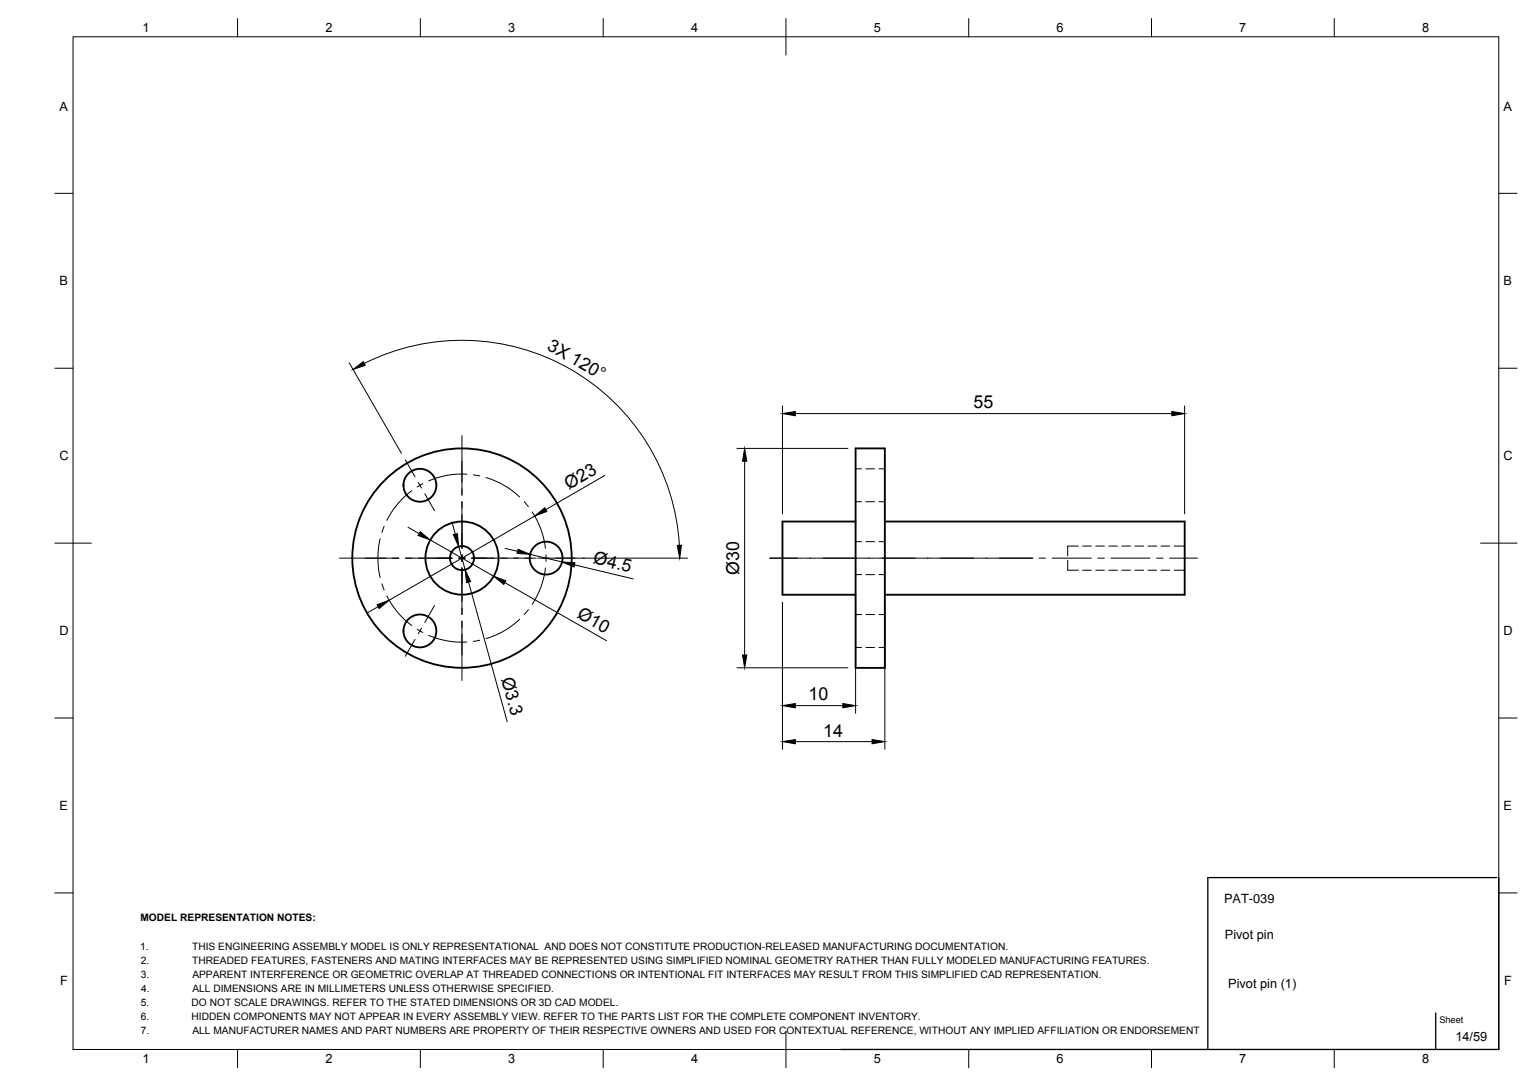
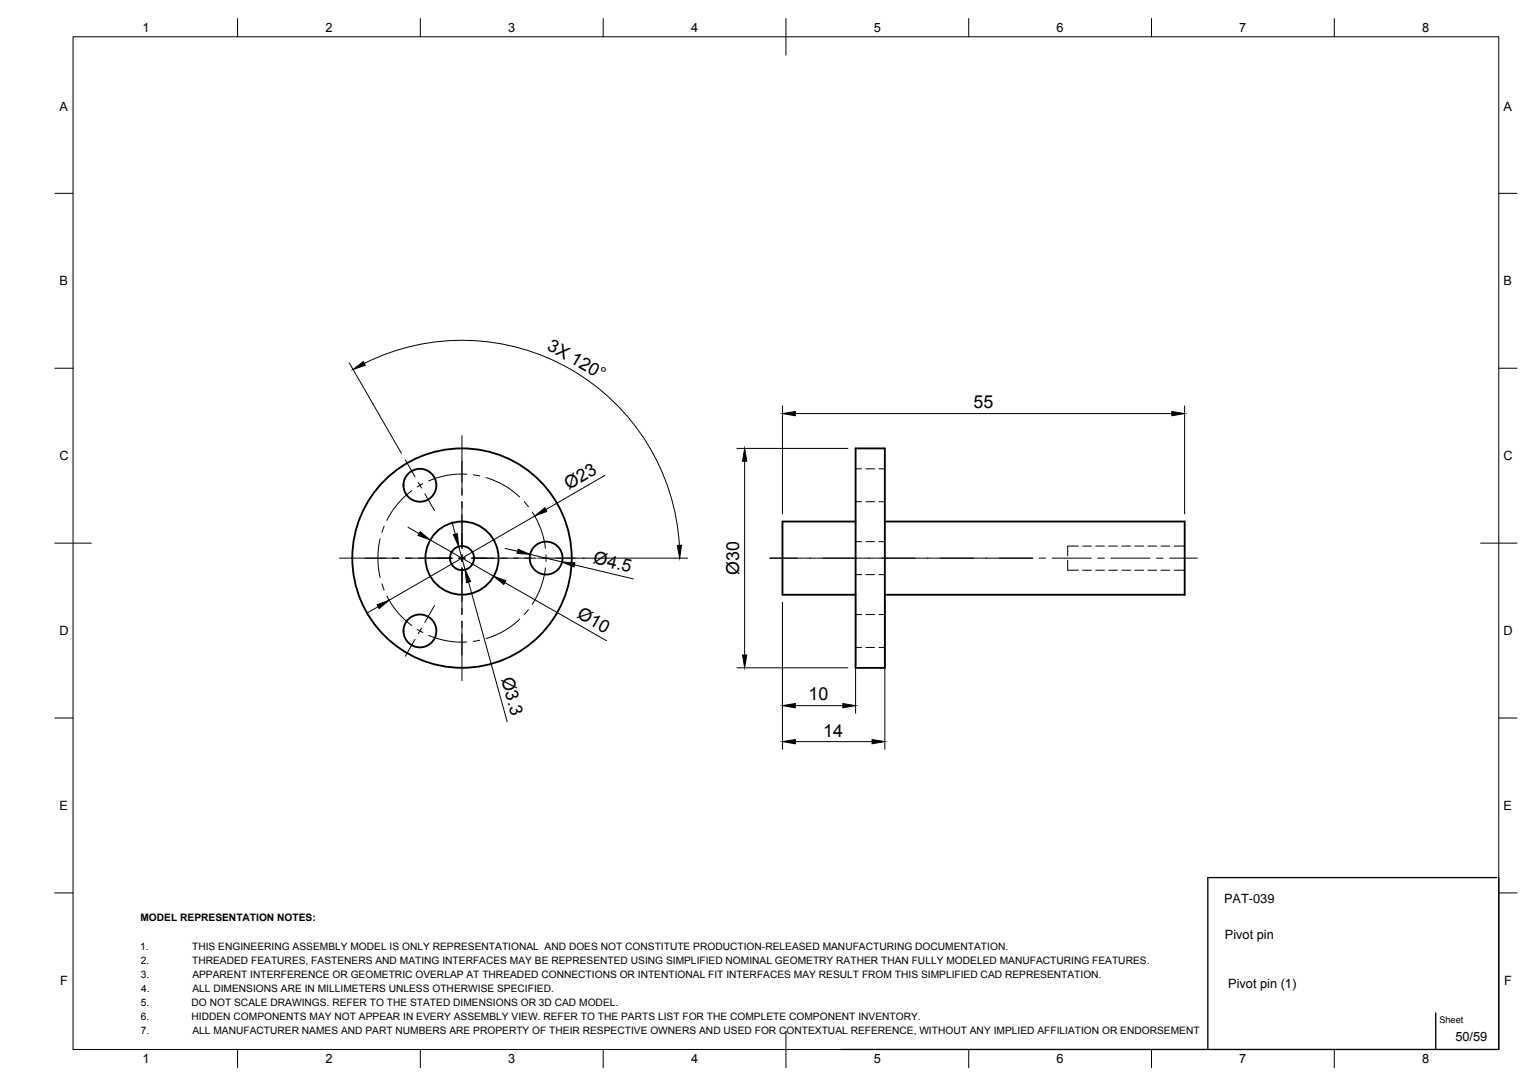
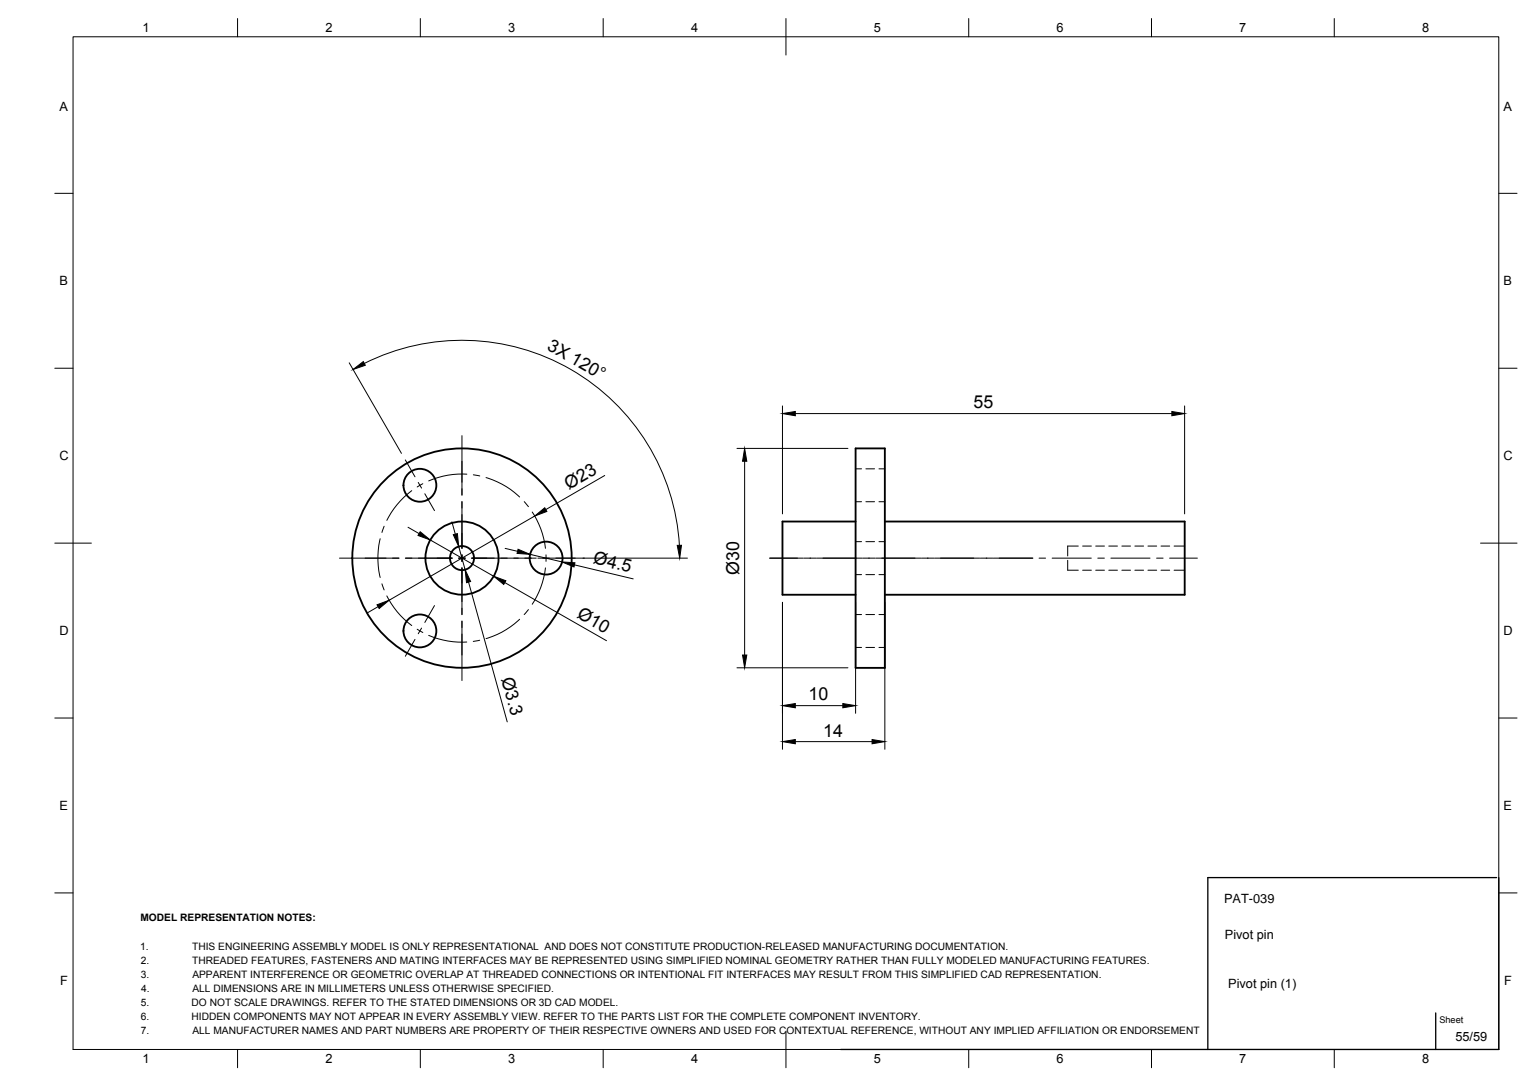
ISO-10303-21;
HEADER;
/* Generated by software containing ST-Developer
 * from STEP Tools, Inc. (www.steptools.com) 
 */

FILE_DESCRIPTION(
/* description */ ('Four-bar parallelogram arm'),
/* implementation_level */ '2;1');

FILE_NAME(
/* name */ 'Pivot pin (1).step',
/* time_stamp */ '2026-10-28T03:24:55-07:00',
/* author */ (''),
/* organization */ (''),
/* preprocessor_version */ 'ST-DEVELOPER v20.2',
/* originating_system */ 'Autodesk Translation Framework v15.17.0.0',
/* authorisation */ '');

FILE_SCHEMA (('AUTOMOTIVE_DESIGN { 1 0 10303 214 3 1 1 }'));
ENDSEC;

DATA;
#10=MECHANICAL_DESIGN_GEOMETRIC_PRESENTATION_REPRESENTATION('',(#669),#14512);
#561=SHAPE_REPRESENTATION_RELATIONSHIP('SRR','None',#14786,#611);
#611=ADVANCED_BREP_SHAPE_REPRESENTATION('',(#725),#14501);
#669=STYLED_ITEM('',(#15087),#725);
#725=MANIFOLD_SOLID_BREP('Body1',#7375);
#971=FACE_BOUND('',#2210,.T.);
#972=FACE_BOUND('',#2211,.T.);
#973=FACE_BOUND('',#2212,.T.);
#974=FACE_BOUND('',#2213,.T.);
#975=FACE_BOUND('',#2215,.T.);
#976=FACE_BOUND('',#2216,.T.);
#977=FACE_BOUND('',#2217,.T.);
#978=FACE_BOUND('',#2218,.T.);
#979=FACE_BOUND('',#2224,.T.);
#1164=PLANE('',#8770);
#1165=PLANE('',#8780);
#1166=PLANE('',#8783);
#1167=PLANE('',#8791);
#1168=PLANE('',#8792);
#1548=FACE_OUTER_BOUND('',#2204,.T.);
#1549=FACE_OUTER_BOUND('',#2205,.T.);
#1550=FACE_OUTER_BOUND('',#2206,.T.);
#1551=FACE_OUTER_BOUND('',#2207,.T.);
#1552=FACE_OUTER_BOUND('',#2208,.T.);
#1553=FACE_OUTER_BOUND('',#2209,.T.);
#1554=FACE_OUTER_BOUND('',#2214,.T.);
#1555=FACE_OUTER_BOUND('',#2219,.T.);
#1556=FACE_OUTER_BOUND('',#2220,.T.);
#1557=FACE_OUTER_BOUND('',#2221,.T.);
#1558=FACE_OUTER_BOUND('',#2222,.T.);
#1559=FACE_OUTER_BOUND('',#2223,.T.);
#2204=EDGE_LOOP('',(#6470,#6471,#6472,#6473));
#2205=EDGE_LOOP('',(#6474));
#2206=EDGE_LOOP('',(#6475,#6476,#6477,#6478));
#2207=EDGE_LOOP('',(#6479,#6480,#6481,#6482));
#2208=EDGE_LOOP('',(#6483,#6484,#6485,#6486));
#2209=EDGE_LOOP('',(#6487));
#2210=EDGE_LOOP('',(#6488));
#2211=EDGE_LOOP('',(#6489));
#2212=EDGE_LOOP('',(#6490));
#2213=EDGE_LOOP('',(#6491));
#2214=EDGE_LOOP('',(#6492));
#2215=EDGE_LOOP('',(#6493));
#2216=EDGE_LOOP('',(#6494));
#2217=EDGE_LOOP('',(#6495));
#2218=EDGE_LOOP('',(#6496));
#2219=EDGE_LOOP('',(#6497,#6498,#6499,#6500));
#2220=EDGE_LOOP('',(#6501,#6502,#6503,#6504));
#2221=EDGE_LOOP('',(#6505,#6506,#6507,#6508));
#2222=EDGE_LOOP('',(#6509));
#2223=EDGE_LOOP('',(#6510));
#2224=EDGE_LOOP('',(#6511));
#2652=LINE('',#14066,#3046);
#2653=LINE('',#14073,#3047);
#2654=LINE('',#14079,#3048);
#2655=LINE('',#14085,#3049);
#2656=LINE('',#14098,#3050);
#2657=LINE('',#14101,#3051);
#2658=LINE('',#14106,#3052);
#3046=VECTOR('',#10972,0.164999999999999);
#3047=VECTOR('',#10981,0.225000000000001);
#3048=VECTOR('',#10988,0.225000000000001);
#3049=VECTOR('',#10995,0.225000000000001);
#3050=VECTOR('',#11012,1.5);
#3051=VECTOR('',#11015,0.5);
#3052=VECTOR('',#11022,0.5);
#3477=CIRCLE('',#8768,0.164999999999999);
#3478=CIRCLE('',#8769,0.164999999999999);
#3479=CIRCLE('',#8772,0.225000000000001);
#3480=CIRCLE('',#8773,0.225000000000001);
#3481=CIRCLE('',#8775,0.225000000000001);
#3482=CIRCLE('',#8776,0.225000000000001);
#3483=CIRCLE('',#8778,0.225000000000001);
#3484=CIRCLE('',#8779,0.225000000000001);
#3485=CIRCLE('',#8781,1.5);
#3486=CIRCLE('',#8782,0.5);
#3487=CIRCLE('',#8784,1.5);
#3488=CIRCLE('',#8785,0.5);
#3489=CIRCLE('',#8788,0.5);
#3490=CIRCLE('',#8790,0.5);
#4045=VERTEX_POINT('',#14063);
#4046=VERTEX_POINT('',#14065);
#4047=VERTEX_POINT('',#14070);
#4048=VERTEX_POINT('',#14072);
#4049=VERTEX_POINT('',#14076);
#4050=VERTEX_POINT('',#14078);
#4051=VERTEX_POINT('',#14082);
#4052=VERTEX_POINT('',#14084);
#4053=VERTEX_POINT('',#14088);
#4054=VERTEX_POINT('',#14090);
#4055=VERTEX_POINT('',#14093);
#4056=VERTEX_POINT('',#14095);
#4057=VERTEX_POINT('',#14100);
#4058=VERTEX_POINT('',#14104);
#4866=EDGE_CURVE('',#4045,#4045,#3477,.T.);
#4867=EDGE_CURVE('',#4045,#4046,#2652,.T.);
#4868=EDGE_CURVE('',#4046,#4046,#3478,.T.);
#4869=EDGE_CURVE('',#4047,#4047,#3479,.T.);
#4870=EDGE_CURVE('',#4047,#4048,#2653,.T.);
#4871=EDGE_CURVE('',#4048,#4048,#3480,.T.);
#4872=EDGE_CURVE('',#4049,#4049,#3481,.T.);
#4873=EDGE_CURVE('',#4049,#4050,#2654,.T.);
#4874=EDGE_CURVE('',#4050,#4050,#3482,.T.);
#4875=EDGE_CURVE('',#4051,#4051,#3483,.T.);
#4876=EDGE_CURVE('',#4051,#4052,#2655,.T.);
#4877=EDGE_CURVE('',#4052,#4052,#3484,.T.);
#4878=EDGE_CURVE('',#4053,#4053,#3485,.T.);
#4879=EDGE_CURVE('',#4054,#4054,#3486,.T.);
#4880=EDGE_CURVE('',#4055,#4055,#3487,.T.);
#4881=EDGE_CURVE('',#4056,#4056,#3488,.T.);
#4882=EDGE_CURVE('',#4053,#4055,#2656,.T.);
#4883=EDGE_CURVE('',#4056,#4057,#2657,.T.);
#4884=EDGE_CURVE('',#4057,#4057,#3489,.T.);
#4885=EDGE_CURVE('',#4058,#4058,#3490,.T.);
#4886=EDGE_CURVE('',#4058,#4054,#2658,.T.);
#6470=ORIENTED_EDGE('',*,*,#4866,.F.);
#6471=ORIENTED_EDGE('',*,*,#4867,.T.);
#6472=ORIENTED_EDGE('',*,*,#4868,.T.);
#6473=ORIENTED_EDGE('',*,*,#4867,.F.);
#6474=ORIENTED_EDGE('',*,*,#4868,.F.);
#6475=ORIENTED_EDGE('',*,*,#4869,.F.);
#6476=ORIENTED_EDGE('',*,*,#4870,.T.);
#6477=ORIENTED_EDGE('',*,*,#4871,.F.);
#6478=ORIENTED_EDGE('',*,*,#4870,.F.);
#6479=ORIENTED_EDGE('',*,*,#4872,.F.);
#6480=ORIENTED_EDGE('',*,*,#4873,.T.);
#6481=ORIENTED_EDGE('',*,*,#4874,.F.);
#6482=ORIENTED_EDGE('',*,*,#4873,.F.);
#6483=ORIENTED_EDGE('',*,*,#4875,.F.);
#6484=ORIENTED_EDGE('',*,*,#4876,.T.);
#6485=ORIENTED_EDGE('',*,*,#4877,.F.);
#6486=ORIENTED_EDGE('',*,*,#4876,.F.);
#6487=ORIENTED_EDGE('',*,*,#4878,.T.);
#6488=ORIENTED_EDGE('',*,*,#4871,.T.);
#6489=ORIENTED_EDGE('',*,*,#4874,.T.);
#6490=ORIENTED_EDGE('',*,*,#4877,.T.);
#6491=ORIENTED_EDGE('',*,*,#4879,.F.);
#6492=ORIENTED_EDGE('',*,*,#4880,.F.);
#6493=ORIENTED_EDGE('',*,*,#4869,.T.);
#6494=ORIENTED_EDGE('',*,*,#4872,.T.);
#6495=ORIENTED_EDGE('',*,*,#4875,.T.);
#6496=ORIENTED_EDGE('',*,*,#4881,.F.);
#6497=ORIENTED_EDGE('',*,*,#4878,.F.);
#6498=ORIENTED_EDGE('',*,*,#4882,.T.);
#6499=ORIENTED_EDGE('',*,*,#4880,.T.);
#6500=ORIENTED_EDGE('',*,*,#4882,.F.);
#6501=ORIENTED_EDGE('',*,*,#4881,.T.);
#6502=ORIENTED_EDGE('',*,*,#4883,.T.);
#6503=ORIENTED_EDGE('',*,*,#4884,.T.);
#6504=ORIENTED_EDGE('',*,*,#4883,.F.);
#6505=ORIENTED_EDGE('',*,*,#4885,.F.);
#6506=ORIENTED_EDGE('',*,*,#4886,.T.);
#6507=ORIENTED_EDGE('',*,*,#4879,.T.);
#6508=ORIENTED_EDGE('',*,*,#4886,.F.);
#6509=ORIENTED_EDGE('',*,*,#4885,.T.);
#6510=ORIENTED_EDGE('',*,*,#4884,.F.);
#6511=ORIENTED_EDGE('',*,*,#4866,.T.);
#6874=CYLINDRICAL_SURFACE('',#8767,0.164999999999999);
#6875=CYLINDRICAL_SURFACE('',#8771,0.225000000000001);
#6876=CYLINDRICAL_SURFACE('',#8774,0.225000000000001);
#6877=CYLINDRICAL_SURFACE('',#8777,0.225000000000001);
#6878=CYLINDRICAL_SURFACE('',#8786,1.5);
#6879=CYLINDRICAL_SURFACE('',#8787,0.5);
#6880=CYLINDRICAL_SURFACE('',#8789,0.5);
#7253=ADVANCED_FACE('',(#1548),#6874,.F.);
#7254=ADVANCED_FACE('',(#1549),#1164,.F.);
#7255=ADVANCED_FACE('',(#1550),#6875,.F.);
#7256=ADVANCED_FACE('',(#1551),#6876,.F.);
#7257=ADVANCED_FACE('',(#1552),#6877,.F.);
#7258=ADVANCED_FACE('',(#1553,#971,#972,#973,#974),#1165,.T.);
#7259=ADVANCED_FACE('',(#1554,#975,#976,#977,#978),#1166,.F.);
#7260=ADVANCED_FACE('',(#1555),#6878,.T.);
#7261=ADVANCED_FACE('',(#1556),#6879,.T.);
#7262=ADVANCED_FACE('',(#1557),#6880,.T.);
#7263=ADVANCED_FACE('',(#1558),#1167,.T.);
#7264=ADVANCED_FACE('',(#1559,#979),#1168,.F.);
#7375=CLOSED_SHELL('',(#7253,#7254,#7255,#7256,#7257,#7258,#7259,#7260,
#7261,#7262,#7263,#7264));
#8766=AXIS2_PLACEMENT_3D('',#14061,#10966,#10967);
#8767=AXIS2_PLACEMENT_3D('',#14062,#10968,#10969);
#8768=AXIS2_PLACEMENT_3D('',#14064,#10970,#10971);
#8769=AXIS2_PLACEMENT_3D('',#14067,#10973,#10974);
#8770=AXIS2_PLACEMENT_3D('',#14068,#10975,#10976);
#8771=AXIS2_PLACEMENT_3D('',#14069,#10977,#10978);
#8772=AXIS2_PLACEMENT_3D('',#14071,#10979,#10980);
#8773=AXIS2_PLACEMENT_3D('',#14074,#10982,#10983);
#8774=AXIS2_PLACEMENT_3D('',#14075,#10984,#10985);
#8775=AXIS2_PLACEMENT_3D('',#14077,#10986,#10987);
#8776=AXIS2_PLACEMENT_3D('',#14080,#10989,#10990);
#8777=AXIS2_PLACEMENT_3D('',#14081,#10991,#10992);
#8778=AXIS2_PLACEMENT_3D('',#14083,#10993,#10994);
#8779=AXIS2_PLACEMENT_3D('',#14086,#10996,#10997);
#8780=AXIS2_PLACEMENT_3D('',#14087,#10998,#10999);
#8781=AXIS2_PLACEMENT_3D('',#14089,#11000,#11001);
#8782=AXIS2_PLACEMENT_3D('',#14091,#11002,#11003);
#8783=AXIS2_PLACEMENT_3D('',#14092,#11004,#11005);
#8784=AXIS2_PLACEMENT_3D('',#14094,#11006,#11007);
#8785=AXIS2_PLACEMENT_3D('',#14096,#11008,#11009);
#8786=AXIS2_PLACEMENT_3D('',#14097,#11010,#11011);
#8787=AXIS2_PLACEMENT_3D('',#14099,#11013,#11014);
#8788=AXIS2_PLACEMENT_3D('',#14102,#11016,#11017);
#8789=AXIS2_PLACEMENT_3D('',#14103,#11018,#11019);
#8790=AXIS2_PLACEMENT_3D('',#14105,#11020,#11021);
#8791=AXIS2_PLACEMENT_3D('',#14107,#11023,#11024);
#8792=AXIS2_PLACEMENT_3D('',#14108,#11025,#11026);
#10966=DIRECTION('axis',(0.,0.,1.));
#10967=DIRECTION('refdir',(1.,0.,0.));
#10968=DIRECTION('center_axis',(0.,1.,0.));
#10969=DIRECTION('ref_axis',(1.,0.,0.));
#10970=DIRECTION('center_axis',(0.,1.,0.));
#10971=DIRECTION('ref_axis',(1.,0.,0.));
#10972=DIRECTION('',(0.,1.,0.));
#10973=DIRECTION('center_axis',(0.,1.,0.));
#10974=DIRECTION('ref_axis',(1.,0.,0.));
#10975=DIRECTION('center_axis',(0.,1.,0.));
#10976=DIRECTION('ref_axis',(1.,0.,0.));
#10977=DIRECTION('center_axis',(0.,1.,0.));
#10978=DIRECTION('ref_axis',(1.,0.,0.));
#10979=DIRECTION('center_axis',(0.,1.,0.));
#10980=DIRECTION('ref_axis',(1.,0.,0.));
#10981=DIRECTION('',(0.,1.,0.));
#10982=DIRECTION('center_axis',(0.,-1.,0.));
#10983=DIRECTION('ref_axis',(1.,0.,0.));
#10984=DIRECTION('center_axis',(0.,1.,0.));
#10985=DIRECTION('ref_axis',(1.,0.,0.));
#10986=DIRECTION('center_axis',(0.,1.,0.));
#10987=DIRECTION('ref_axis',(1.,0.,0.));
#10988=DIRECTION('',(0.,1.,0.));
#10989=DIRECTION('center_axis',(0.,-1.,0.));
#10990=DIRECTION('ref_axis',(1.,0.,0.));
#10991=DIRECTION('center_axis',(0.,1.,0.));
#10992=DIRECTION('ref_axis',(1.,0.,0.));
#10993=DIRECTION('center_axis',(0.,1.,0.));
#10994=DIRECTION('ref_axis',(1.,0.,0.));
#10995=DIRECTION('',(0.,1.,0.));
#10996=DIRECTION('center_axis',(0.,-1.,0.));
#10997=DIRECTION('ref_axis',(1.,0.,0.));
#10998=DIRECTION('center_axis',(0.,1.,0.));
#10999=DIRECTION('ref_axis',(1.,0.,0.));
#11000=DIRECTION('center_axis',(0.,1.,0.));
#11001=DIRECTION('ref_axis',(1.,0.,0.));
#11002=DIRECTION('center_axis',(0.,1.,0.));
#11003=DIRECTION('ref_axis',(1.,0.,0.));
#11004=DIRECTION('center_axis',(0.,1.,0.));
#11005=DIRECTION('ref_axis',(1.,0.,0.));
#11006=DIRECTION('center_axis',(0.,1.,0.));
#11007=DIRECTION('ref_axis',(1.,0.,0.));
#11008=DIRECTION('center_axis',(0.,-1.,0.));
#11009=DIRECTION('ref_axis',(1.,0.,0.));
#11010=DIRECTION('center_axis',(0.,1.,0.));
#11011=DIRECTION('ref_axis',(1.,0.,0.));
#11012=DIRECTION('',(0.,-1.,0.));
#11013=DIRECTION('center_axis',(0.,1.,0.));
#11014=DIRECTION('ref_axis',(1.,0.,0.));
#11015=DIRECTION('',(0.,-1.,0.));
#11016=DIRECTION('center_axis',(0.,1.,0.));
#11017=DIRECTION('ref_axis',(1.,0.,0.));
#11018=DIRECTION('center_axis',(0.,1.,0.));
#11019=DIRECTION('ref_axis',(1.,0.,0.));
#11020=DIRECTION('center_axis',(0.,1.,0.));
#11021=DIRECTION('ref_axis',(1.,0.,0.));
#11022=DIRECTION('',(0.,-1.,0.));
#11023=DIRECTION('center_axis',(0.,1.,0.));
#11024=DIRECTION('ref_axis',(1.,0.,0.));
#11025=DIRECTION('center_axis',(0.,1.,0.));
#11026=DIRECTION('ref_axis',(1.,0.,0.));
#14061=CARTESIAN_POINT('',(0.,0.,0.));
#14062=CARTESIAN_POINT('Origin',(20.,-1.7,8.));
#14063=CARTESIAN_POINT('',(19.835,-1.6,8.));
#14064=CARTESIAN_POINT('Origin',(20.,-1.6,8.));
#14065=CARTESIAN_POINT('',(19.835,0.,8.));
#14066=CARTESIAN_POINT('',(19.835,-1.7,8.));
#14067=CARTESIAN_POINT('Origin',(20.,0.,8.));
#14068=CARTESIAN_POINT('Origin',(20.,0.,8.));
#14069=CARTESIAN_POINT('Origin',(21.15,2.4,8.));
#14070=CARTESIAN_POINT('',(20.925,2.5,8.));
#14071=CARTESIAN_POINT('Origin',(21.15,2.5,8.));
#14072=CARTESIAN_POINT('',(20.925,2.9,8.));
#14073=CARTESIAN_POINT('',(20.925,2.4,8.));
#14074=CARTESIAN_POINT('Origin',(21.15,2.9,8.));
#14075=CARTESIAN_POINT('Origin',(19.425,2.4,8.9959292143521));
#14076=CARTESIAN_POINT('',(19.2,2.5,8.9959292143521));
#14077=CARTESIAN_POINT('Origin',(19.425,2.5,8.9959292143521));
#14078=CARTESIAN_POINT('',(19.2,2.9,8.9959292143521));
#14079=CARTESIAN_POINT('',(19.2,2.4,8.9959292143521));
#14080=CARTESIAN_POINT('Origin',(19.425,2.9,8.9959292143521));
#14081=CARTESIAN_POINT('Origin',(19.425,2.4,7.0040707856479));
#14082=CARTESIAN_POINT('',(19.2,2.5,7.0040707856479));
#14083=CARTESIAN_POINT('Origin',(19.425,2.5,7.0040707856479));
#14084=CARTESIAN_POINT('',(19.2,2.9,7.0040707856479));
#14085=CARTESIAN_POINT('',(19.2,2.4,7.0040707856479));
#14086=CARTESIAN_POINT('Origin',(19.425,2.9,7.0040707856479));
#14087=CARTESIAN_POINT('Origin',(20.,2.9,8.));
#14088=CARTESIAN_POINT('',(18.5,2.9,8.));
#14089=CARTESIAN_POINT('Origin',(20.,2.9,8.));
#14090=CARTESIAN_POINT('',(19.5,2.9,8.));
#14091=CARTESIAN_POINT('Origin',(20.,2.9,8.));
#14092=CARTESIAN_POINT('Origin',(20.,2.5,8.));
#14093=CARTESIAN_POINT('',(18.5,2.5,8.));
#14094=CARTESIAN_POINT('Origin',(20.,2.5,8.));
#14095=CARTESIAN_POINT('',(19.5,2.5,8.));
#14096=CARTESIAN_POINT('Origin',(20.,2.5,8.));
#14097=CARTESIAN_POINT('Origin',(20.,2.5,8.));
#14098=CARTESIAN_POINT('',(18.5,2.5,8.));
#14099=CARTESIAN_POINT('Origin',(20.,-1.6,8.));
#14100=CARTESIAN_POINT('',(19.5,-1.6,8.));
#14101=CARTESIAN_POINT('',(19.5,-1.6,8.));
#14102=CARTESIAN_POINT('Origin',(20.,-1.6,8.));
#14103=CARTESIAN_POINT('Origin',(20.,-1.6,8.));
#14104=CARTESIAN_POINT('',(19.5,3.9,8.));
#14105=CARTESIAN_POINT('Origin',(20.,3.9,8.));
#14106=CARTESIAN_POINT('',(19.5,-1.6,8.));
#14107=CARTESIAN_POINT('Origin',(20.,3.9,8.));
#14108=CARTESIAN_POINT('Origin',(20.,-1.6,8.));
#14444=UNCERTAINTY_MEASURE_WITH_UNIT(LENGTH_MEASURE(0.001),#14513,
'DISTANCE_ACCURACY_VALUE',
'Maximum model space distance between geometric entities at asserted c
onnectivities');
#14455=UNCERTAINTY_MEASURE_WITH_UNIT(LENGTH_MEASURE(0.001),#14513,
'DISTANCE_ACCURACY_VALUE',
'Maximum model space distance between geometric entities at asserted c
onnectivities');
#14501=(
GEOMETRIC_REPRESENTATION_CONTEXT(3)
GLOBAL_UNCERTAINTY_ASSIGNED_CONTEXT((#14444))
GLOBAL_UNIT_ASSIGNED_CONTEXT((#14513,#14515,#14516))
REPRESENTATION_CONTEXT('','3D')
);
#14512=(
GEOMETRIC_REPRESENTATION_CONTEXT(3)
GLOBAL_UNCERTAINTY_ASSIGNED_CONTEXT((#14455))
GLOBAL_UNIT_ASSIGNED_CONTEXT((#14513,#14515,#14516))
REPRESENTATION_CONTEXT('','3D')
);
#14513=(
LENGTH_UNIT()
NAMED_UNIT(*)
SI_UNIT(.CENTI.,.METRE.)
);
#14515=(
NAMED_UNIT(*)
PLANE_ANGLE_UNIT()
SI_UNIT($,.RADIAN.)
);
#14516=(
NAMED_UNIT(*)
SI_UNIT($,.STERADIAN.)
SOLID_ANGLE_UNIT()
);
#14562=SHAPE_DEFINITION_REPRESENTATION(#14678,#14786);
#14678=PRODUCT_DEFINITION_SHAPE('',$,#14843);
#14786=SHAPE_REPRESENTATION('',(#8766),#14501);
#14797=PRODUCT_DEFINITION_CONTEXT('part definition',#14967,'design');
#14843=PRODUCT_DEFINITION('Pivot pin (1)','Pivot pin (1)',#14899,#14797);
#14899=PRODUCT_DEFINITION_FORMATION('',$,#15014);
#14967=APPLICATION_CONTEXT(
'Core Data for Automotive Mechanical Design Process');
#14968=PRODUCT_CONTEXT('part definition',#14967,'mechanical');
#15014=PRODUCT('Pivot pin (1)','Pivot pin (1)','Pivot pin (1)',(#14968));
#15081=COLOUR_RGB('Grey',0.48,0.52,0.57);
#15082=FILL_AREA_STYLE_COLOUR('',#15081);
#15083=FILL_AREA_STYLE('',(#15082));
#15084=SURFACE_STYLE_FILL_AREA(#15083);
#15085=SURFACE_SIDE_STYLE('',(#15084));
#15086=SURFACE_STYLE_USAGE(.BOTH.,#15085);
#15087=PRESENTATION_STYLE_ASSIGNMENT((#15086));
ENDSEC;
END-ISO-10303-21;
